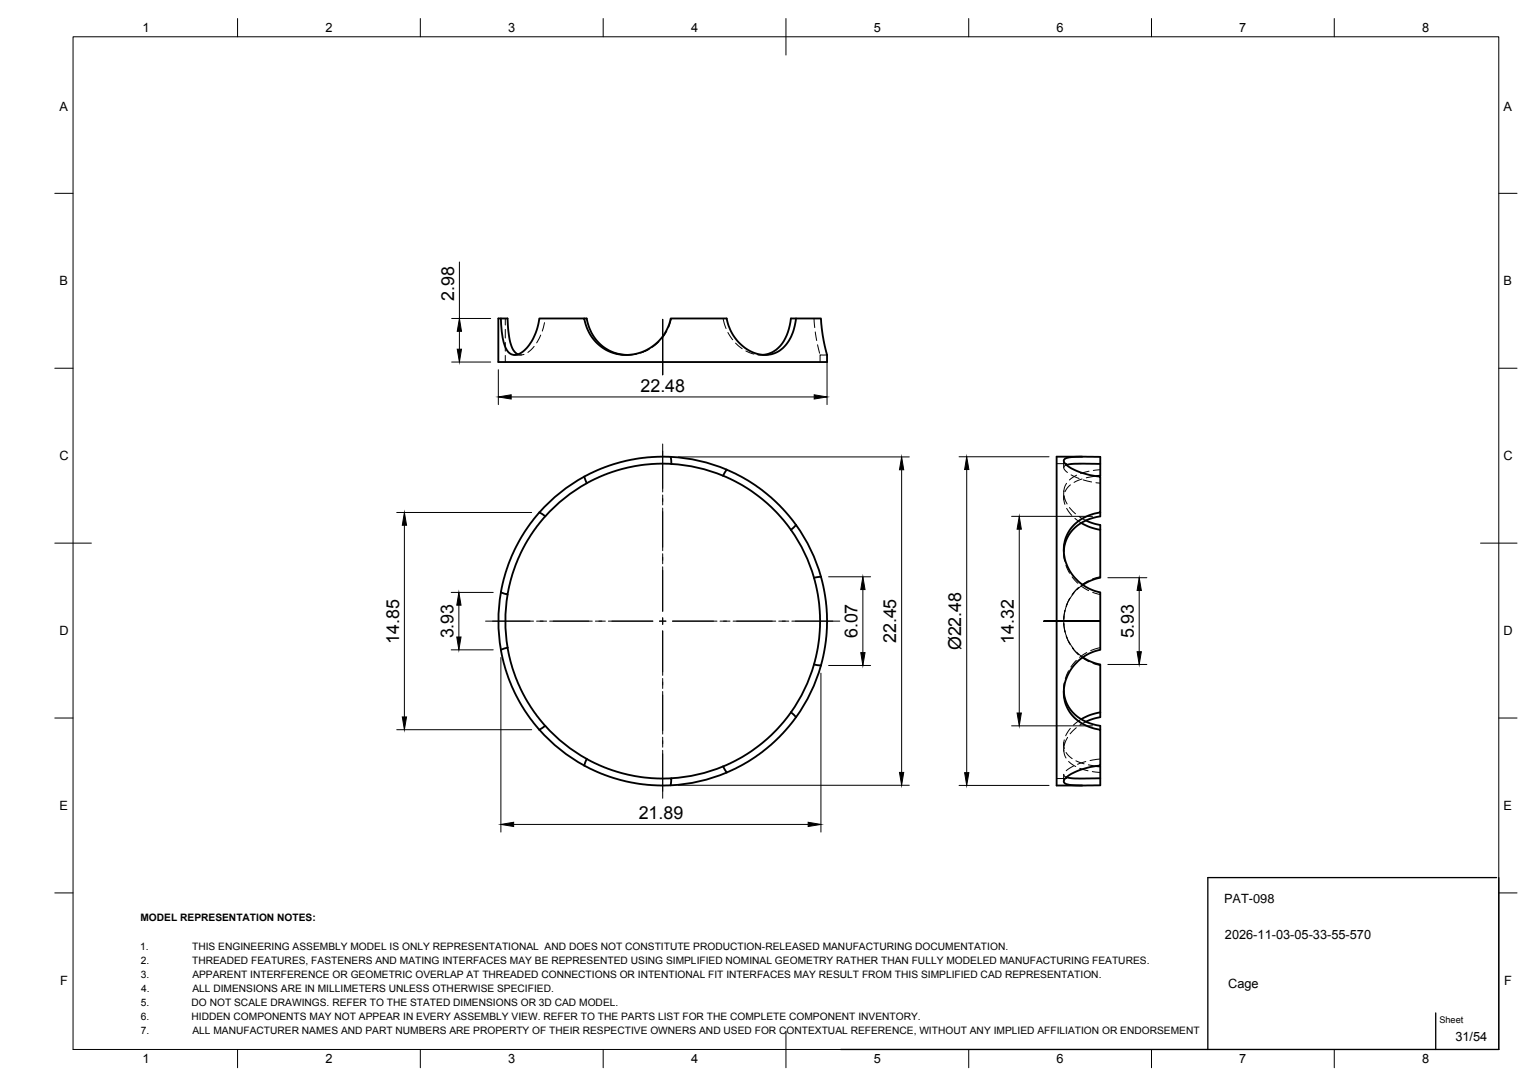
ISO-10303-21;
HEADER;
/* Generated by software containing ST-Developer
 * from STEP Tools, Inc. (www.steptools.com) 
 */

FILE_DESCRIPTION(
/* description */ ('Spring compression tester'),
/* implementation_level */ '2;1');

FILE_NAME(
/* name */ 'Cage.step',
/* time_stamp */ '2026-10-28T03:24:11-07:00',
/* author */ (''),
/* organization */ (''),
/* preprocessor_version */ 'ST-DEVELOPER v20.2',
/* originating_system */ 'Autodesk Translation Framework v15.17.0.0',
/* authorisation */ '');

FILE_SCHEMA (('AUTOMOTIVE_DESIGN { 1 0 10303 214 3 1 1 }'));
ENDSEC;

DATA;
#10=MECHANICAL_DESIGN_GEOMETRIC_PRESENTATION_REPRESENTATION('',(#1136),#43521);
#553=B_SPLINE_CURVE_WITH_KNOTS('',3,(#28592,#28593,#28594,#28595,#28596,
#28597,#28598,#28599,#28600,#28601,#28602,#28603,#28604,#28605,#28606,#28607,
#28608,#28609,#28610,#28611,#28612,#28613),.UNSPECIFIED.,.F.,.F.,(4,2,2,
2,2,2,2,2,2,2,4),(0.0591825211272536,0.157966726598481,0.236950089897721,
0.315933453196962,0.391576304923761,0.46721915665056,0.54286200837736,0.618504860104159,
0.697488223403399,0.77647158670264,0.875255792173867),.UNSPECIFIED.);
#554=B_SPLINE_CURVE_WITH_KNOTS('',3,(#28617,#28618,#28619,#28620,#28621,
#28622,#28623,#28624,#28625,#28626,#28627,#28628,#28629,#28630,#28631,#28632,
#28633,#28634,#28635,#28636,#28637,#28638),.UNSPECIFIED.,.F.,.F.,(4,2,2,
2,2,2,2,2,2,2,4),(0.0581119756758434,0.106553146291161,0.213106292582322,
0.30849933801665,0.386091982889075,0.4636846277615,0.541277272633925,0.61886991750635,
0.714262962940678,0.820816109231839,0.869257279847157),.UNSPECIFIED.);
#555=B_SPLINE_CURVE_WITH_KNOTS('',3,(#28644,#28645,#28646,#28647,#28648,
#28649,#28650,#28651,#28652,#28653,#28654,#28655,#28656,#28657,#28658,#28659,
#28660,#28661,#28662,#28663,#28664,#28665),.UNSPECIFIED.,.F.,.F.,(4,2,2,
2,2,2,2,2,2,2,4),(0.0581119756758434,0.106553146291161,0.213106292582322,
0.30849933801665,0.386091982889075,0.4636846277615,0.541277272633925,0.61886991750635,
0.714262962940679,0.820816109231839,0.869257279847157),.UNSPECIFIED.);
#556=B_SPLINE_CURVE_WITH_KNOTS('',3,(#28669,#28670,#28671,#28672,#28673,
#28674,#28675,#28676,#28677,#28678,#28679,#28680,#28681,#28682,#28683,#28684,
#28685,#28686,#28687,#28688,#28689,#28690),.UNSPECIFIED.,.F.,.F.,(4,2,2,
2,2,2,2,2,2,2,4),(0.0581119756758433,0.106553146291161,0.213106292582322,
0.308499338016649,0.386091982889075,0.4636846277615,0.541277272633925,0.61886991750635,
0.714262962940678,0.820816109231839,0.869257279847157),.UNSPECIFIED.);
#557=B_SPLINE_CURVE_WITH_KNOTS('',3,(#28699,#28700,#28701,#28702,#28703,
#28704,#28705,#28706,#28707,#28708,#28709,#28710,#28711,#28712,#28713,#28714,
#28715,#28716,#28717,#28718,#28719,#28720),.UNSPECIFIED.,.F.,.F.,(4,2,2,
2,2,2,2,2,2,2,4),(0.0581119756758433,0.106553146291161,0.213106292582322,
0.30849933801665,0.386091982889075,0.4636846277615,0.541277272633925,0.61886991750635,
0.714262962940678,0.820816109231839,0.869257279847157),.UNSPECIFIED.);
#558=B_SPLINE_CURVE_WITH_KNOTS('',3,(#28724,#28725,#28726,#28727,#28728,
#28729,#28730,#28731,#28732,#28733,#28734,#28735,#28736,#28737,#28738,#28739,
#28740,#28741,#28742,#28743,#28744,#28745),.UNSPECIFIED.,.F.,.F.,(4,2,2,
2,2,2,2,2,2,2,4),(0.0581119756758434,0.106553146291161,0.213106292582322,
0.30849933801665,0.386091982889075,0.4636846277615,0.541277272633925,0.61886991750635,
0.714262962940678,0.820816109231839,0.869257279847157),.UNSPECIFIED.);
#559=B_SPLINE_CURVE_WITH_KNOTS('',3,(#28749,#28750,#28751,#28752,#28753,
#28754,#28755,#28756,#28757,#28758,#28759,#28760,#28761,#28762,#28763,#28764,
#28765,#28766,#28767,#28768,#28769,#28770),.UNSPECIFIED.,.F.,.F.,(4,2,2,
2,2,2,2,2,2,2,4),(0.0581119756758434,0.106553146291161,0.213106292582322,
0.30849933801665,0.386091982889075,0.4636846277615,0.541277272633925,0.61886991750635,
0.714262962940678,0.820816109231839,0.869257279847157),.UNSPECIFIED.);
#560=B_SPLINE_CURVE_WITH_KNOTS('',3,(#28774,#28775,#28776,#28777,#28778,
#28779,#28780,#28781,#28782,#28783,#28784,#28785,#28786,#28787,#28788,#28789,
#28790,#28791,#28792,#28793,#28794,#28795),.UNSPECIFIED.,.F.,.F.,(4,2,2,
2,2,2,2,2,2,2,4),(0.0581119756758433,0.106553146291161,0.213106292582322,
0.30849933801665,0.386091982889075,0.4636846277615,0.541277272633925,0.61886991750635,
0.714262962940678,0.820816109231839,0.869257279847157),.UNSPECIFIED.);
#561=B_SPLINE_CURVE_WITH_KNOTS('',3,(#28803,#28804,#28805,#28806,#28807,
#28808,#28809,#28810,#28811,#28812,#28813,#28814,#28815,#28816,#28817,#28818,
#28819,#28820,#28821,#28822,#28823,#28824),.UNSPECIFIED.,.F.,.F.,(4,2,2,
2,2,2,2,2,2,2,4),(0.0591825211272536,0.157966726598481,0.236950089897721,
0.315933453196962,0.391576304923761,0.467219156650561,0.54286200837736,
0.618504860104159,0.697488223403399,0.77647158670264,0.875255792173867),
 .UNSPECIFIED.);
#562=B_SPLINE_CURVE_WITH_KNOTS('',3,(#28832,#28833,#28834,#28835,#28836,
#28837,#28838,#28839,#28840,#28841,#28842,#28843,#28844,#28845,#28846,#28847,
#28848,#28849,#28850,#28851,#28852,#28853),.UNSPECIFIED.,.F.,.F.,(4,2,2,
2,2,2,2,2,2,2,4),(0.0591825211272536,0.157966726598481,0.236950089897722,
0.315933453196962,0.391576304923761,0.467219156650561,0.54286200837736,
0.618504860104159,0.697488223403399,0.77647158670264,0.875255792173867),
 .UNSPECIFIED.);
#563=B_SPLINE_CURVE_WITH_KNOTS('',3,(#28863,#28864,#28865,#28866,#28867,
#28868,#28869,#28870,#28871,#28872,#28873,#28874,#28875,#28876,#28877,#28878,
#28879,#28880,#28881,#28882,#28883,#28884),.UNSPECIFIED.,.F.,.F.,(4,2,2,
2,2,2,2,2,2,2,4),(0.0591825211272536,0.157966726598481,0.236950089897721,
0.315933453196962,0.391576304923761,0.46721915665056,0.54286200837736,0.618504860104159,
0.697488223403399,0.77647158670264,0.875255792173867),.UNSPECIFIED.);
#564=B_SPLINE_CURVE_WITH_KNOTS('',3,(#28892,#28893,#28894,#28895,#28896,
#28897,#28898,#28899,#28900,#28901,#28902,#28903,#28904,#28905,#28906,#28907,
#28908,#28909,#28910,#28911,#28912,#28913),.UNSPECIFIED.,.F.,.F.,(4,2,2,
2,2,2,2,2,2,2,4),(0.0591825211272536,0.157966726598481,0.236950089897721,
0.315933453196962,0.391576304923761,0.46721915665056,0.542862008377359,
0.618504860104159,0.697488223403399,0.776471586702639,0.875255792173867),
 .UNSPECIFIED.);
#565=B_SPLINE_CURVE_WITH_KNOTS('',3,(#28921,#28922,#28923,#28924,#28925,
#28926,#28927,#28928,#28929,#28930,#28931,#28932,#28933,#28934,#28935,#28936,
#28937,#28938,#28939,#28940,#28941,#28942),.UNSPECIFIED.,.F.,.F.,(4,2,2,
2,2,2,2,2,2,2,4),(0.0591825211272536,0.157966726598481,0.236950089897721,
0.315933453196962,0.391576304923761,0.46721915665056,0.54286200837736,0.618504860104159,
0.697488223403399,0.77647158670264,0.875255792173867),.UNSPECIFIED.);
#566=B_SPLINE_CURVE_WITH_KNOTS('',3,(#28951,#28952,#28953,#28954,#28955,
#28956,#28957,#28958,#28959,#28960,#28961,#28962,#28963,#28964,#28965,#28966,
#28967,#28968,#28969,#28970,#28971,#28972),.UNSPECIFIED.,.F.,.F.,(4,2,2,
2,2,2,2,2,2,2,4),(0.0591825211272536,0.157966726598481,0.236950089897721,
0.315933453196962,0.391576304923761,0.46721915665056,0.542862008377359,
0.618504860104159,0.697488223403399,0.776471586702639,0.875255792173867),
 .UNSPECIFIED.);
#904=SPHERICAL_SURFACE('',#20049,0.309556);
#905=SPHERICAL_SURFACE('',#20065,0.309556);
#906=SPHERICAL_SURFACE('',#20070,0.309556);
#907=SPHERICAL_SURFACE('',#20076,0.309556);
#908=SPHERICAL_SURFACE('',#20081,0.309556);
#909=SPHERICAL_SURFACE('',#20086,0.309556);
#910=SPHERICAL_SURFACE('',#20094,0.309556);
#1010=SHAPE_REPRESENTATION_RELATIONSHIP('SRR','None',#43823,#1070);
#1070=ADVANCED_BREP_SHAPE_REPRESENTATION('',(#1210),#43483);
#1136=STYLED_ITEM('',(#44202),#1210);
#1210=MANIFOLD_SOLID_BREP('Continuous crown cage',#18574);
#1454=FACE_BOUND('',#3889,.T.);
#1892=PLANE('',#20062);
#1893=PLANE('',#20067);
#1894=PLANE('',#20072);
#1895=PLANE('',#20078);
#1896=PLANE('',#20083);
#1897=PLANE('',#20092);
#1898=PLANE('',#20096);
#1899=PLANE('',#20097);
#2619=FACE_OUTER_BOUND('',#3873,.T.);
#2620=FACE_OUTER_BOUND('',#3874,.T.);
#2621=FACE_OUTER_BOUND('',#3875,.T.);
#2622=FACE_OUTER_BOUND('',#3876,.T.);
#2623=FACE_OUTER_BOUND('',#3877,.T.);
#2624=FACE_OUTER_BOUND('',#3878,.T.);
#2625=FACE_OUTER_BOUND('',#3879,.T.);
#2626=FACE_OUTER_BOUND('',#3880,.T.);
#2627=FACE_OUTER_BOUND('',#3881,.T.);
#2628=FACE_OUTER_BOUND('',#3882,.T.);
#2629=FACE_OUTER_BOUND('',#3883,.T.);
#2630=FACE_OUTER_BOUND('',#3884,.T.);
#2631=FACE_OUTER_BOUND('',#3885,.T.);
#2632=FACE_OUTER_BOUND('',#3886,.T.);
#2633=FACE_OUTER_BOUND('',#3887,.T.);
#2634=FACE_OUTER_BOUND('',#3888,.T.);
#2635=FACE_OUTER_BOUND('',#3890,.T.);
#3873=EDGE_LOOP('',(#14199,#14200,#14201,#14202));
#3874=EDGE_LOOP('',(#14203,#14204,#14205,#14206,#14207,#14208,#14209,#14210,
#14211,#14212,#14213,#14214,#14215,#14216,#14217,#14218,#14219,#14220));
#3875=EDGE_LOOP('',(#14221,#14222,#14223,#14224));
#3876=EDGE_LOOP('',(#14225,#14226,#14227,#14228));
#3877=EDGE_LOOP('',(#14229,#14230,#14231,#14232));
#3878=EDGE_LOOP('',(#14233,#14234,#14235,#14236));
#3879=EDGE_LOOP('',(#14237,#14238,#14239,#14240,#14241,#14242));
#3880=EDGE_LOOP('',(#14243,#14244,#14245,#14246));
#3881=EDGE_LOOP('',(#14247,#14248,#14249,#14250));
#3882=EDGE_LOOP('',(#14251,#14252,#14253,#14254));
#3883=EDGE_LOOP('',(#14255,#14256,#14257,#14258));
#3884=EDGE_LOOP('',(#14259,#14260,#14261,#14262));
#3885=EDGE_LOOP('',(#14263,#14264,#14265,#14266,#14267,#14268,#14269,#14270,
#14271,#14272,#14273,#14274,#14275,#14276,#14277,#14278,#14279,#14280));
#3886=EDGE_LOOP('',(#14281,#14282,#14283,#14284));
#3887=EDGE_LOOP('',(#14285,#14286,#14287,#14288));
#3888=EDGE_LOOP('',(#14289));
#3889=EDGE_LOOP('',(#14290));
#3890=EDGE_LOOP('',(#14291,#14292,#14293,#14294));
#5311=LINE('',#28694,#6743);
#5312=LINE('',#28947,#6744);
#6743=VECTOR('',#23445,1.123812);
#6744=VECTOR('',#23514,1.076188);
#7756=CIRCLE('',#20050,0.303778037777585);
#7757=CIRCLE('',#20051,0.303778037777585);
#7758=CIRCLE('',#20053,1.123812);
#7759=CIRCLE('',#20054,1.123812);
#7760=CIRCLE('',#20055,1.123812);
#7761=CIRCLE('',#20056,1.123812);
#7762=CIRCLE('',#20057,1.123812);
#7763=CIRCLE('',#20058,1.123812);
#7764=CIRCLE('',#20059,1.123812);
#7765=CIRCLE('',#20060,1.123812);
#7766=CIRCLE('',#20061,1.123812);
#7767=CIRCLE('',#20063,1.076188);
#7768=CIRCLE('',#20064,0.303778037777585);
#7769=CIRCLE('',#20066,0.303778037777585);
#7770=CIRCLE('',#20068,1.076188);
#7771=CIRCLE('',#20069,0.303778037777585);
#7772=CIRCLE('',#20071,0.303778037777585);
#7773=CIRCLE('',#20073,1.076188);
#7774=CIRCLE('',#20074,1.076188);
#7775=CIRCLE('',#20075,0.303778037777585);
#7776=CIRCLE('',#20077,0.303778037777585);
#7777=CIRCLE('',#20079,1.076188);
#7778=CIRCLE('',#20080,0.303778037777585);
#7779=CIRCLE('',#20082,0.303778037777585);
#7780=CIRCLE('',#20084,1.076188);
#7781=CIRCLE('',#20085,0.303778037777585);
#7782=CIRCLE('',#20087,0.303778037777585);
#7783=CIRCLE('',#20089,1.076188);
#7784=CIRCLE('',#20090,1.076188);
#7785=CIRCLE('',#20091,1.076188);
#7786=CIRCLE('',#20093,0.303778037777585);
#7787=CIRCLE('',#20095,0.303778037777585);
#8803=VERTEX_POINT('',#28590);
#8804=VERTEX_POINT('',#28591);
#8805=VERTEX_POINT('',#28614);
#8806=VERTEX_POINT('',#28616);
#8807=VERTEX_POINT('',#28641);
#8808=VERTEX_POINT('',#28643);
#8809=VERTEX_POINT('',#28666);
#8810=VERTEX_POINT('',#28668);
#8811=VERTEX_POINT('',#28691);
#8812=VERTEX_POINT('',#28693);
#8813=VERTEX_POINT('',#28696);
#8814=VERTEX_POINT('',#28698);
#8815=VERTEX_POINT('',#28721);
#8816=VERTEX_POINT('',#28723);
#8817=VERTEX_POINT('',#28746);
#8818=VERTEX_POINT('',#28748);
#8819=VERTEX_POINT('',#28771);
#8820=VERTEX_POINT('',#28773);
#8821=VERTEX_POINT('',#28798);
#8822=VERTEX_POINT('',#28802);
#8823=VERTEX_POINT('',#28827);
#8824=VERTEX_POINT('',#28831);
#8825=VERTEX_POINT('',#28856);
#8826=VERTEX_POINT('',#28858);
#8827=VERTEX_POINT('',#28862);
#8828=VERTEX_POINT('',#28887);
#8829=VERTEX_POINT('',#28891);
#8830=VERTEX_POINT('',#28916);
#8831=VERTEX_POINT('',#28920);
#8832=VERTEX_POINT('',#28945);
#8833=VERTEX_POINT('',#28948);
#8834=VERTEX_POINT('',#28950);
#10764=EDGE_CURVE('',#8803,#8804,#553,.T.);
#10765=EDGE_CURVE('',#8805,#8803,#7756,.T.);
#10766=EDGE_CURVE('',#8806,#8805,#554,.T.);
#10767=EDGE_CURVE('',#8804,#8806,#7757,.T.);
#10768=EDGE_CURVE('',#8807,#8805,#7758,.T.);
#10769=EDGE_CURVE('',#8807,#8808,#555,.T.);
#10770=EDGE_CURVE('',#8809,#8808,#7759,.T.);
#10771=EDGE_CURVE('',#8809,#8810,#556,.T.);
#10772=EDGE_CURVE('',#8811,#8810,#7760,.T.);
#10773=EDGE_CURVE('',#8811,#8812,#5311,.T.);
#10774=EDGE_CURVE('',#8812,#8812,#7761,.T.);
#10775=EDGE_CURVE('',#8813,#8811,#7762,.T.);
#10776=EDGE_CURVE('',#8813,#8814,#557,.T.);
#10777=EDGE_CURVE('',#8815,#8814,#7763,.T.);
#10778=EDGE_CURVE('',#8815,#8816,#558,.T.);
#10779=EDGE_CURVE('',#8817,#8816,#7764,.T.);
#10780=EDGE_CURVE('',#8817,#8818,#559,.T.);
#10781=EDGE_CURVE('',#8819,#8818,#7765,.T.);
#10782=EDGE_CURVE('',#8819,#8820,#560,.T.);
#10783=EDGE_CURVE('',#8806,#8820,#7766,.T.);
#10784=EDGE_CURVE('',#8803,#8821,#7767,.T.);
#10785=EDGE_CURVE('',#8821,#8807,#7768,.T.);
#10786=EDGE_CURVE('',#8822,#8821,#561,.T.);
#10787=EDGE_CURVE('',#8808,#8822,#7769,.T.);
#10788=EDGE_CURVE('',#8822,#8823,#7770,.T.);
#10789=EDGE_CURVE('',#8823,#8809,#7771,.T.);
#10790=EDGE_CURVE('',#8824,#8823,#562,.T.);
#10791=EDGE_CURVE('',#8810,#8824,#7772,.T.);
#10792=EDGE_CURVE('',#8824,#8825,#7773,.T.);
#10793=EDGE_CURVE('',#8825,#8826,#7774,.T.);
#10794=EDGE_CURVE('',#8826,#8813,#7775,.T.);
#10795=EDGE_CURVE('',#8827,#8826,#563,.T.);
#10796=EDGE_CURVE('',#8814,#8827,#7776,.T.);
#10797=EDGE_CURVE('',#8827,#8828,#7777,.T.);
#10798=EDGE_CURVE('',#8828,#8815,#7778,.T.);
#10799=EDGE_CURVE('',#8829,#8828,#564,.T.);
#10800=EDGE_CURVE('',#8816,#8829,#7779,.T.);
#10801=EDGE_CURVE('',#8829,#8830,#7780,.T.);
#10802=EDGE_CURVE('',#8830,#8817,#7781,.T.);
#10803=EDGE_CURVE('',#8831,#8830,#565,.T.);
#10804=EDGE_CURVE('',#8818,#8831,#7782,.T.);
#10805=EDGE_CURVE('',#8832,#8832,#7783,.T.);
#10806=EDGE_CURVE('',#8832,#8825,#5312,.T.);
#10807=EDGE_CURVE('',#8833,#8804,#7784,.T.);
#10808=EDGE_CURVE('',#8833,#8834,#566,.T.);
#10809=EDGE_CURVE('',#8831,#8834,#7785,.T.);
#10810=EDGE_CURVE('',#8820,#8833,#7786,.T.);
#10811=EDGE_CURVE('',#8834,#8819,#7787,.T.);
#14199=ORIENTED_EDGE('',*,*,#10764,.F.);
#14200=ORIENTED_EDGE('',*,*,#10765,.F.);
#14201=ORIENTED_EDGE('',*,*,#10766,.F.);
#14202=ORIENTED_EDGE('',*,*,#10767,.F.);
#14203=ORIENTED_EDGE('',*,*,#10766,.T.);
#14204=ORIENTED_EDGE('',*,*,#10768,.F.);
#14205=ORIENTED_EDGE('',*,*,#10769,.T.);
#14206=ORIENTED_EDGE('',*,*,#10770,.F.);
#14207=ORIENTED_EDGE('',*,*,#10771,.T.);
#14208=ORIENTED_EDGE('',*,*,#10772,.F.);
#14209=ORIENTED_EDGE('',*,*,#10773,.T.);
#14210=ORIENTED_EDGE('',*,*,#10774,.F.);
#14211=ORIENTED_EDGE('',*,*,#10773,.F.);
#14212=ORIENTED_EDGE('',*,*,#10775,.F.);
#14213=ORIENTED_EDGE('',*,*,#10776,.T.);
#14214=ORIENTED_EDGE('',*,*,#10777,.F.);
#14215=ORIENTED_EDGE('',*,*,#10778,.T.);
#14216=ORIENTED_EDGE('',*,*,#10779,.F.);
#14217=ORIENTED_EDGE('',*,*,#10780,.T.);
#14218=ORIENTED_EDGE('',*,*,#10781,.F.);
#14219=ORIENTED_EDGE('',*,*,#10782,.T.);
#14220=ORIENTED_EDGE('',*,*,#10783,.F.);
#14221=ORIENTED_EDGE('',*,*,#10765,.T.);
#14222=ORIENTED_EDGE('',*,*,#10784,.T.);
#14223=ORIENTED_EDGE('',*,*,#10785,.T.);
#14224=ORIENTED_EDGE('',*,*,#10768,.T.);
#14225=ORIENTED_EDGE('',*,*,#10786,.F.);
#14226=ORIENTED_EDGE('',*,*,#10787,.F.);
#14227=ORIENTED_EDGE('',*,*,#10769,.F.);
#14228=ORIENTED_EDGE('',*,*,#10785,.F.);
#14229=ORIENTED_EDGE('',*,*,#10787,.T.);
#14230=ORIENTED_EDGE('',*,*,#10788,.T.);
#14231=ORIENTED_EDGE('',*,*,#10789,.T.);
#14232=ORIENTED_EDGE('',*,*,#10770,.T.);
#14233=ORIENTED_EDGE('',*,*,#10790,.F.);
#14234=ORIENTED_EDGE('',*,*,#10791,.F.);
#14235=ORIENTED_EDGE('',*,*,#10771,.F.);
#14236=ORIENTED_EDGE('',*,*,#10789,.F.);
#14237=ORIENTED_EDGE('',*,*,#10791,.T.);
#14238=ORIENTED_EDGE('',*,*,#10792,.T.);
#14239=ORIENTED_EDGE('',*,*,#10793,.T.);
#14240=ORIENTED_EDGE('',*,*,#10794,.T.);
#14241=ORIENTED_EDGE('',*,*,#10775,.T.);
#14242=ORIENTED_EDGE('',*,*,#10772,.T.);
#14243=ORIENTED_EDGE('',*,*,#10795,.F.);
#14244=ORIENTED_EDGE('',*,*,#10796,.F.);
#14245=ORIENTED_EDGE('',*,*,#10776,.F.);
#14246=ORIENTED_EDGE('',*,*,#10794,.F.);
#14247=ORIENTED_EDGE('',*,*,#10796,.T.);
#14248=ORIENTED_EDGE('',*,*,#10797,.T.);
#14249=ORIENTED_EDGE('',*,*,#10798,.T.);
#14250=ORIENTED_EDGE('',*,*,#10777,.T.);
#14251=ORIENTED_EDGE('',*,*,#10799,.F.);
#14252=ORIENTED_EDGE('',*,*,#10800,.F.);
#14253=ORIENTED_EDGE('',*,*,#10778,.F.);
#14254=ORIENTED_EDGE('',*,*,#10798,.F.);
#14255=ORIENTED_EDGE('',*,*,#10800,.T.);
#14256=ORIENTED_EDGE('',*,*,#10801,.T.);
#14257=ORIENTED_EDGE('',*,*,#10802,.T.);
#14258=ORIENTED_EDGE('',*,*,#10779,.T.);
#14259=ORIENTED_EDGE('',*,*,#10780,.F.);
#14260=ORIENTED_EDGE('',*,*,#10802,.F.);
#14261=ORIENTED_EDGE('',*,*,#10803,.F.);
#14262=ORIENTED_EDGE('',*,*,#10804,.F.);
#14263=ORIENTED_EDGE('',*,*,#10805,.F.);
#14264=ORIENTED_EDGE('',*,*,#10806,.T.);
#14265=ORIENTED_EDGE('',*,*,#10792,.F.);
#14266=ORIENTED_EDGE('',*,*,#10790,.T.);
#14267=ORIENTED_EDGE('',*,*,#10788,.F.);
#14268=ORIENTED_EDGE('',*,*,#10786,.T.);
#14269=ORIENTED_EDGE('',*,*,#10784,.F.);
#14270=ORIENTED_EDGE('',*,*,#10764,.T.);
#14271=ORIENTED_EDGE('',*,*,#10807,.F.);
#14272=ORIENTED_EDGE('',*,*,#10808,.T.);
#14273=ORIENTED_EDGE('',*,*,#10809,.F.);
#14274=ORIENTED_EDGE('',*,*,#10803,.T.);
#14275=ORIENTED_EDGE('',*,*,#10801,.F.);
#14276=ORIENTED_EDGE('',*,*,#10799,.T.);
#14277=ORIENTED_EDGE('',*,*,#10797,.F.);
#14278=ORIENTED_EDGE('',*,*,#10795,.T.);
#14279=ORIENTED_EDGE('',*,*,#10793,.F.);
#14280=ORIENTED_EDGE('',*,*,#10806,.F.);
#14281=ORIENTED_EDGE('',*,*,#10767,.T.);
#14282=ORIENTED_EDGE('',*,*,#10783,.T.);
#14283=ORIENTED_EDGE('',*,*,#10810,.T.);
#14284=ORIENTED_EDGE('',*,*,#10807,.T.);
#14285=ORIENTED_EDGE('',*,*,#10782,.F.);
#14286=ORIENTED_EDGE('',*,*,#10811,.F.);
#14287=ORIENTED_EDGE('',*,*,#10808,.F.);
#14288=ORIENTED_EDGE('',*,*,#10810,.F.);
#14289=ORIENTED_EDGE('',*,*,#10774,.T.);
#14290=ORIENTED_EDGE('',*,*,#10805,.T.);
#14291=ORIENTED_EDGE('',*,*,#10804,.T.);
#14292=ORIENTED_EDGE('',*,*,#10809,.T.);
#14293=ORIENTED_EDGE('',*,*,#10811,.T.);
#14294=ORIENTED_EDGE('',*,*,#10781,.T.);
#17233=CYLINDRICAL_SURFACE('',#20052,1.123812);
#17234=CYLINDRICAL_SURFACE('',#20088,1.076188);
#17943=ADVANCED_FACE('',(#2619),#904,.F.);
#17944=ADVANCED_FACE('',(#2620),#17233,.T.);
#17945=ADVANCED_FACE('',(#2621),#1892,.T.);
#17946=ADVANCED_FACE('',(#2622),#905,.F.);
#17947=ADVANCED_FACE('',(#2623),#1893,.T.);
#17948=ADVANCED_FACE('',(#2624),#906,.F.);
#17949=ADVANCED_FACE('',(#2625),#1894,.T.);
#17950=ADVANCED_FACE('',(#2626),#907,.F.);
#17951=ADVANCED_FACE('',(#2627),#1895,.T.);
#17952=ADVANCED_FACE('',(#2628),#908,.F.);
#17953=ADVANCED_FACE('',(#2629),#1896,.T.);
#17954=ADVANCED_FACE('',(#2630),#909,.F.);
#17955=ADVANCED_FACE('',(#2631),#17234,.F.);
#17956=ADVANCED_FACE('',(#2632),#1897,.T.);
#17957=ADVANCED_FACE('',(#2633),#910,.F.);
#17958=ADVANCED_FACE('',(#2634,#1454),#1898,.T.);
#17959=ADVANCED_FACE('',(#2635),#1899,.T.);
#18574=CLOSED_SHELL('',(#17943,#17944,#17945,#17946,#17947,#17948,#17949,
#17950,#17951,#17952,#17953,#17954,#17955,#17956,#17957,#17958,#17959));
#20048=AXIS2_PLACEMENT_3D('',#28588,#23429,#23430);
#20049=AXIS2_PLACEMENT_3D('',#28589,#23431,#23432);
#20050=AXIS2_PLACEMENT_3D('',#28615,#23433,#23434);
#20051=AXIS2_PLACEMENT_3D('',#28639,#23435,#23436);
#20052=AXIS2_PLACEMENT_3D('',#28640,#23437,#23438);
#20053=AXIS2_PLACEMENT_3D('',#28642,#23439,#23440);
#20054=AXIS2_PLACEMENT_3D('',#28667,#23441,#23442);
#20055=AXIS2_PLACEMENT_3D('',#28692,#23443,#23444);
#20056=AXIS2_PLACEMENT_3D('',#28695,#23446,#23447);
#20057=AXIS2_PLACEMENT_3D('',#28697,#23448,#23449);
#20058=AXIS2_PLACEMENT_3D('',#28722,#23450,#23451);
#20059=AXIS2_PLACEMENT_3D('',#28747,#23452,#23453);
#20060=AXIS2_PLACEMENT_3D('',#28772,#23454,#23455);
#20061=AXIS2_PLACEMENT_3D('',#28796,#23456,#23457);
#20062=AXIS2_PLACEMENT_3D('',#28797,#23458,#23459);
#20063=AXIS2_PLACEMENT_3D('',#28799,#23460,#23461);
#20064=AXIS2_PLACEMENT_3D('',#28800,#23462,#23463);
#20065=AXIS2_PLACEMENT_3D('',#28801,#23464,#23465);
#20066=AXIS2_PLACEMENT_3D('',#28825,#23466,#23467);
#20067=AXIS2_PLACEMENT_3D('',#28826,#23468,#23469);
#20068=AXIS2_PLACEMENT_3D('',#28828,#23470,#23471);
#20069=AXIS2_PLACEMENT_3D('',#28829,#23472,#23473);
#20070=AXIS2_PLACEMENT_3D('',#28830,#23474,#23475);
#20071=AXIS2_PLACEMENT_3D('',#28854,#23476,#23477);
#20072=AXIS2_PLACEMENT_3D('',#28855,#23478,#23479);
#20073=AXIS2_PLACEMENT_3D('',#28857,#23480,#23481);
#20074=AXIS2_PLACEMENT_3D('',#28859,#23482,#23483);
#20075=AXIS2_PLACEMENT_3D('',#28860,#23484,#23485);
#20076=AXIS2_PLACEMENT_3D('',#28861,#23486,#23487);
#20077=AXIS2_PLACEMENT_3D('',#28885,#23488,#23489);
#20078=AXIS2_PLACEMENT_3D('',#28886,#23490,#23491);
#20079=AXIS2_PLACEMENT_3D('',#28888,#23492,#23493);
#20080=AXIS2_PLACEMENT_3D('',#28889,#23494,#23495);
#20081=AXIS2_PLACEMENT_3D('',#28890,#23496,#23497);
#20082=AXIS2_PLACEMENT_3D('',#28914,#23498,#23499);
#20083=AXIS2_PLACEMENT_3D('',#28915,#23500,#23501);
#20084=AXIS2_PLACEMENT_3D('',#28917,#23502,#23503);
#20085=AXIS2_PLACEMENT_3D('',#28918,#23504,#23505);
#20086=AXIS2_PLACEMENT_3D('',#28919,#23506,#23507);
#20087=AXIS2_PLACEMENT_3D('',#28943,#23508,#23509);
#20088=AXIS2_PLACEMENT_3D('',#28944,#23510,#23511);
#20089=AXIS2_PLACEMENT_3D('',#28946,#23512,#23513);
#20090=AXIS2_PLACEMENT_3D('',#28949,#23515,#23516);
#20091=AXIS2_PLACEMENT_3D('',#28973,#23517,#23518);
#20092=AXIS2_PLACEMENT_3D('',#28974,#23519,#23520);
#20093=AXIS2_PLACEMENT_3D('',#28975,#23521,#23522);
#20094=AXIS2_PLACEMENT_3D('',#28976,#23523,#23524);
#20095=AXIS2_PLACEMENT_3D('',#28977,#23525,#23526);
#20096=AXIS2_PLACEMENT_3D('',#28978,#23527,#23528);
#20097=AXIS2_PLACEMENT_3D('',#28979,#23529,#23530);
#23429=DIRECTION('axis',(0.,0.,1.));
#23430=DIRECTION('refdir',(1.,0.,0.));
#23431=DIRECTION('center_axis',(0.,0.,1.));
#23432=DIRECTION('ref_axis',(1.,0.,0.));
#23433=DIRECTION('center_axis',(0.,-1.,0.));
#23434=DIRECTION('ref_axis',(0.,0.,-1.));
#23435=DIRECTION('center_axis',(0.,-1.,0.));
#23436=DIRECTION('ref_axis',(0.,0.,-1.));
#23437=DIRECTION('center_axis',(0.,1.,0.));
#23438=DIRECTION('ref_axis',(1.,0.,0.));
#23439=DIRECTION('center_axis',(0.,1.,0.));
#23440=DIRECTION('ref_axis',(1.,0.,0.));
#23441=DIRECTION('center_axis',(0.,1.,0.));
#23442=DIRECTION('ref_axis',(1.,0.,0.));
#23443=DIRECTION('center_axis',(0.,1.,0.));
#23444=DIRECTION('ref_axis',(1.,0.,0.));
#23445=DIRECTION('',(0.,-1.,0.));
#23446=DIRECTION('center_axis',(0.,-1.,0.));
#23447=DIRECTION('ref_axis',(1.,0.,0.));
#23448=DIRECTION('center_axis',(0.,1.,0.));
#23449=DIRECTION('ref_axis',(1.,0.,0.));
#23450=DIRECTION('center_axis',(0.,1.,0.));
#23451=DIRECTION('ref_axis',(1.,0.,0.));
#23452=DIRECTION('center_axis',(0.,1.,0.));
#23453=DIRECTION('ref_axis',(1.,0.,0.));
#23454=DIRECTION('center_axis',(0.,1.,0.));
#23455=DIRECTION('ref_axis',(1.,0.,0.));
#23456=DIRECTION('center_axis',(0.,1.,0.));
#23457=DIRECTION('ref_axis',(1.,0.,0.));
#23458=DIRECTION('center_axis',(0.,1.,0.));
#23459=DIRECTION('ref_axis',(1.,0.,0.));
#23460=DIRECTION('center_axis',(0.,-1.,0.));
#23461=DIRECTION('ref_axis',(1.,0.,0.));
#23462=DIRECTION('center_axis',(0.,-1.,0.));
#23463=DIRECTION('ref_axis',(0.,0.,-1.));
#23464=DIRECTION('center_axis',(8.96625347776458E-17,0.,1.));
#23465=DIRECTION('ref_axis',(1.,0.,0.));
#23466=DIRECTION('center_axis',(0.,-1.,0.));
#23467=DIRECTION('ref_axis',(0.,0.,-1.));
#23468=DIRECTION('center_axis',(0.,1.,0.));
#23469=DIRECTION('ref_axis',(1.,0.,0.));
#23470=DIRECTION('center_axis',(0.,-1.,0.));
#23471=DIRECTION('ref_axis',(1.,0.,0.));
#23472=DIRECTION('center_axis',(0.,-1.,0.));
#23473=DIRECTION('ref_axis',(0.,0.,-1.));
#23474=DIRECTION('center_axis',(0.,0.,1.));
#23475=DIRECTION('ref_axis',(1.,0.,0.));
#23476=DIRECTION('center_axis',(0.,-1.,0.));
#23477=DIRECTION('ref_axis',(0.,0.,-1.));
#23478=DIRECTION('center_axis',(0.,1.,0.));
#23479=DIRECTION('ref_axis',(1.,0.,0.));
#23480=DIRECTION('center_axis',(0.,-1.,0.));
#23481=DIRECTION('ref_axis',(1.,0.,0.));
#23482=DIRECTION('center_axis',(0.,-1.,0.));
#23483=DIRECTION('ref_axis',(1.,0.,0.));
#23484=DIRECTION('center_axis',(0.,-1.,0.));
#23485=DIRECTION('ref_axis',(0.,0.,-1.));
#23486=DIRECTION('center_axis',(0.,0.,1.));
#23487=DIRECTION('ref_axis',(1.,0.,0.));
#23488=DIRECTION('center_axis',(0.,-1.,0.));
#23489=DIRECTION('ref_axis',(0.,0.,-1.));
#23490=DIRECTION('center_axis',(0.,1.,0.));
#23491=DIRECTION('ref_axis',(1.,0.,0.));
#23492=DIRECTION('center_axis',(0.,-1.,0.));
#23493=DIRECTION('ref_axis',(1.,0.,0.));
#23494=DIRECTION('center_axis',(0.,-1.,0.));
#23495=DIRECTION('ref_axis',(0.,0.,-1.));
#23496=DIRECTION('center_axis',(8.96625347776458E-17,0.,1.));
#23497=DIRECTION('ref_axis',(1.,0.,0.));
#23498=DIRECTION('center_axis',(0.,-1.,0.));
#23499=DIRECTION('ref_axis',(0.,0.,-1.));
#23500=DIRECTION('center_axis',(0.,1.,0.));
#23501=DIRECTION('ref_axis',(1.,0.,0.));
#23502=DIRECTION('center_axis',(0.,-1.,0.));
#23503=DIRECTION('ref_axis',(1.,0.,0.));
#23504=DIRECTION('center_axis',(0.,-1.,0.));
#23505=DIRECTION('ref_axis',(0.,0.,-1.));
#23506=DIRECTION('center_axis',(0.,0.,1.));
#23507=DIRECTION('ref_axis',(1.,0.,0.));
#23508=DIRECTION('center_axis',(0.,-1.,0.));
#23509=DIRECTION('ref_axis',(0.,0.,-1.));
#23510=DIRECTION('center_axis',(0.,1.,0.));
#23511=DIRECTION('ref_axis',(1.,0.,0.));
#23512=DIRECTION('center_axis',(0.,1.,0.));
#23513=DIRECTION('ref_axis',(1.,0.,0.));
#23514=DIRECTION('',(0.,1.,0.));
#23515=DIRECTION('center_axis',(0.,-1.,0.));
#23516=DIRECTION('ref_axis',(1.,0.,0.));
#23517=DIRECTION('center_axis',(0.,-1.,0.));
#23518=DIRECTION('ref_axis',(1.,0.,0.));
#23519=DIRECTION('center_axis',(0.,1.,0.));
#23520=DIRECTION('ref_axis',(1.,0.,0.));
#23521=DIRECTION('center_axis',(0.,-1.,0.));
#23522=DIRECTION('ref_axis',(0.,0.,-1.));
#23523=DIRECTION('center_axis',(0.,0.,1.));
#23524=DIRECTION('ref_axis',(1.,0.,0.));
#23525=DIRECTION('center_axis',(0.,-1.,0.));
#23526=DIRECTION('ref_axis',(0.,0.,-1.));
#23527=DIRECTION('center_axis',(0.,-1.,0.));
#23528=DIRECTION('ref_axis',(-1.,0.,0.));
#23529=DIRECTION('center_axis',(0.,1.,0.));
#23530=DIRECTION('ref_axis',(1.,0.,0.));
#28588=CARTESIAN_POINT('',(0.,0.,0.));
#28589=CARTESIAN_POINT('Origin',(0.685838782044607,0.,0.860014630714833));
#28590=CARTESIAN_POINT('',(0.413083465285518,-0.05953,0.993751811093549));
#28591=CARTESIAN_POINT('',(0.876916659919095,-0.05953,0.623857181492959));
#28592=CARTESIAN_POINT('Ctrl Pts',(0.413083465285518,-0.05953,0.993751811093549));
#28593=CARTESIAN_POINT('Ctrl Pts',(0.419070565453383,-0.0925528133349865,
0.991263089003441));
#28594=CARTESIAN_POINT('Ctrl Pts',(0.430199341854858,-0.124911173756694,
0.986608710139579));
#28595=CARTESIAN_POINT('Ctrl Pts',(0.457978755888596,-0.177924977804098,
0.973971221090534));
#28596=CARTESIAN_POINT('Ctrl Pts',(0.473077587363685,-0.199697230012983,
0.966820759530997));
#28597=CARTESIAN_POINT('Ctrl Pts',(0.507057380724533,-0.237895043532788,
0.949440676105255));
#28598=CARTESIAN_POINT('Ctrl Pts',(0.525933334162555,-0.254319232363049,
0.939198248544428));
#28599=CARTESIAN_POINT('Ctrl Pts',(0.564362943424238,-0.28018331644634,
0.916597376014514));
#28600=CARTESIAN_POINT('Ctrl Pts',(0.585840553788742,-0.29104845371857,
0.903141581680914));
#28601=CARTESIAN_POINT('Ctrl Pts',(0.629305439856167,-0.30527573347708,
0.873412008702649));
#28602=CARTESIAN_POINT('Ctrl Pts',(0.651278921914856,-0.308638795020976,
0.857118508332695));
#28603=CARTESIAN_POINT('Ctrl Pts',(0.690705563850638,-0.308638795020976,
0.825676810575914));
#28604=CARTESIAN_POINT('Ctrl Pts',(0.711480111898423,-0.30527573347708,
0.807879894508811));
#28605=CARTESIAN_POINT('Ctrl Pts',(0.750136149454208,-0.29104845371857,
0.772120216227122));
#28606=CARTESIAN_POINT('Ctrl Pts',(0.768033796848072,-0.28018331644634,
0.754175290318038));
#28607=CARTESIAN_POINT('Ctrl Pts',(0.798619410861634,-0.254319232363049,
0.721738358858166));
#28608=CARTESIAN_POINT('Ctrl Pts',(0.812805334167529,-0.237895043532788,
0.705614819529209));
#28609=CARTESIAN_POINT('Ctrl Pts',(0.837310877969633,-0.199697230012983,
0.676354402927683));
#28610=CARTESIAN_POINT('Ctrl Pts',(0.847641868610495,-0.177924977804098,
0.663225258065736));
#28611=CARTESIAN_POINT('Ctrl Pts',(0.866144010579847,-0.124911173756694,
0.638954437806245));
#28612=CARTESIAN_POINT('Ctrl Pts',(0.873158080166742,-0.0925528133349865,
0.62914037979579));
#28613=CARTESIAN_POINT('Ctrl Pts',(0.876916659919095,-0.05953,0.623857181492959));
#28614=CARTESIAN_POINT('',(0.437601487681057,-0.05953,1.03511272300331));
#28615=CARTESIAN_POINT('Origin',(0.685838782044607,-0.05953,0.860014630714833));
#28616=CARTESIAN_POINT('',(0.911784794170997,-0.05953,0.656964154625313));
#28617=CARTESIAN_POINT('Ctrl Pts',(0.911784794170998,-0.0595300000000001,
0.656964154625312));
#28618=CARTESIAN_POINT('Ctrl Pts',(0.909827729890942,-0.0762225747374255,
0.659680317203144));
#28619=CARTESIAN_POINT('Ctrl Pts',(0.907004864562642,-0.0928409665394228,
0.663576540841106));
#28620=CARTESIAN_POINT('Ctrl Pts',(0.895234408667242,-0.144299303100741,
0.679480524217551));
#28621=CARTESIAN_POINT('Ctrl Pts',(0.882797231409153,-0.177024326825049,
0.695831250979106));
#28622=CARTESIAN_POINT('Ctrl Pts',(0.854332839576145,-0.227269801620064,
0.73042219438957));
#28623=CARTESIAN_POINT('Ctrl Pts',(0.834863020612702,-0.251265615809407,
0.752807465209441));
#28624=CARTESIAN_POINT('Ctrl Pts',(0.800439809856111,-0.279889827963178,
0.789147407129766));
#28625=CARTESIAN_POINT('Ctrl Pts',(0.781998747691871,-0.290879136862659,
0.80756613568454));
#28626=CARTESIAN_POINT('Ctrl Pts',(0.742239891936898,-0.305251990234487,
0.844254137480382));
#28627=CARTESIAN_POINT('Ctrl Pts',(0.720906778729541,-0.308638795020976,
0.862505527716294));
#28628=CARTESIAN_POINT('Ctrl Pts',(0.680463863683392,-0.308638795020976,
0.894757676234429));
#28629=CARTESIAN_POINT('Ctrl Pts',(0.657923009631182,-0.305251990234488,
0.91149460735272));
#28630=CARTESIAN_POINT('Ctrl Pts',(0.613307674922609,-0.290879136862659,
0.942092777160053));
#28631=CARTESIAN_POINT('Ctrl Pts',(0.591247219971725,-0.279889827963178,
0.955972930713954));
#28632=CARTESIAN_POINT('Ctrl Pts',(0.548158511259202,-0.251265615809407,
0.981446681891443));
#28633=CARTESIAN_POINT('Ctrl Pts',(0.522002043615455,-0.227269801620063,
0.995447160474328));
#28634=CARTESIAN_POINT('Ctrl Pts',(0.481944444320713,-0.177024326825049,
1.01550068154148));
#28635=CARTESIAN_POINT('Ctrl Pts',(0.463236132117164,-0.14429930310074,
1.0239876538093));
#28636=CARTESIAN_POINT('Ctrl Pts',(0.445111721969657,-0.0928409665394226,
1.03192403056628));
#28637=CARTESIAN_POINT('Ctrl Pts',(0.440685038163619,-0.0762225747374254,
1.03380912944435));
#28638=CARTESIAN_POINT('Ctrl Pts',(0.437601487681056,-0.05953,1.03511272300331));
#28639=CARTESIAN_POINT('Origin',(0.685838782044607,-0.05953,0.860014630714833));
#28640=CARTESIAN_POINT('Origin',(0.,-0.208355,0.));
#28641=CARTESIAN_POINT('',(0.0548532617164168,-0.05953,1.12247250791415));
#28642=CARTESIAN_POINT('Origin',(0.,-0.05953,0.));
#28643=CARTESIAN_POINT('',(-0.536443649899848,-0.05953,0.987512846410683));
#28644=CARTESIAN_POINT('Ctrl Pts',(0.0548532617164173,-0.0595300000000001,
1.12247250791414));
#28645=CARTESIAN_POINT('Ctrl Pts',(0.05150947068137,-0.0762225747374254,
1.12263591311425));
#28646=CARTESIAN_POINT('Ctrl Pts',(0.0467032526342597,-0.0928409665394227,
1.12285816383385));
#28647=CARTESIAN_POINT('Ctrl Pts',(0.0269302585198975,-0.144299303100741,
1.12357162229597));
#28648=CARTESIAN_POINT('Ctrl Pts',(0.006392292392153,-0.177024326825049,
1.12404235695137));
#28649=CARTESIAN_POINT('Ctrl Pts',(-0.0383992541984087,-0.227269801620063,
1.12335509974011));
#28650=CARTESIAN_POINT('Ctrl Pts',(-0.0680399972366993,-0.251265615809407,
1.12208997038458));
#28651=CARTESIAN_POINT('Ctrl Pts',(-0.117914228755037,-0.279889827963178,
1.1178344036749));
#28652=CARTESIAN_POINT('Ctrl Pts',(-0.14381238480104,-0.290879136862659,
1.11490049012186));
#28653=CARTESIAN_POINT('Ctrl Pts',(-0.19728546073067,-0.305251990234488,
1.10669035995599));
#28654=CARTESIAN_POINT('Ctrl Pts',(-0.224855950742601,-0.308638795020976,
1.10139101611326));
#28655=CARTESIAN_POINT('Ctrl Pts',(-0.275287440920027,-0.308638795020976,
1.0898803575765));
#28656=CARTESIAN_POINT('Ctrl Pts',(-0.302426893214945,-0.305251990234488,
1.08269251410343));
#28657=CARTESIAN_POINT('Ctrl Pts',(-0.35416671187353,-0.290879136862659,
1.06688848765783));
#28658=CARTESIAN_POINT('Ctrl Pts',(-0.3787731215897,-0.279889827963178,
1.05829506364875));
#28659=CARTESIAN_POINT('Ctrl Pts',(-0.425554672694338,-0.251265615809407,
1.04048957871266));
#28660=CARTESIAN_POINT('Ctrl Pts',(-0.452808978448581,-0.227269801620063,
1.02876878445619));
#28661=CARTESIAN_POINT('Ctrl Pts',(-0.493462957200432,-0.177024326825049,
1.0099536580922));
#28662=CARTESIAN_POINT('Ctrl Pts',(-0.511762781179148,-0.14429930310074,
1.00061845128527));
#28663=CARTESIAN_POINT('Ctrl Pts',(-0.529268075276157,-0.0928409665394226,
0.991396466802468));
#28664=CARTESIAN_POINT('Ctrl Pts',(-0.533501897135713,-0.0762225747374254,
0.989110885965947));
#28665=CARTESIAN_POINT('Ctrl Pts',(-0.536443649899848,-0.0595300000000001,
0.987512846410683));
#28666=CARTESIAN_POINT('',(-0.843383895613249,-0.05953,0.742736168477219));
#28667=CARTESIAN_POINT('Origin',(0.,-0.05953,0.));
#28668=CARTESIAN_POINT('',(-1.10653577764992,-0.05953,0.196295654879792));
#28669=CARTESIAN_POINT('Ctrl Pts',(-0.843383895613249,-0.0595300000000001,
0.742736168477219));
#28670=CARTESIAN_POINT('Ctrl Pts',(-0.84559647055299,-0.0762225747374255,
0.740223768851062));
#28671=CARTESIAN_POINT('Ctrl Pts',(-0.848766861100456,-0.0928409665394227,
0.736604687327351));
#28672=CARTESIAN_POINT('Ctrl Pts',(-0.861652925570091,-0.144299303100741,
0.721590372101268));
#28673=CARTESIAN_POINT('Ctrl Pts',(-0.87482617317514,-0.177024326825049,
0.705826641853758));
#28674=CARTESIAN_POINT('Ctrl Pts',(-0.902215926359523,-0.227269801620063,
0.670378702718353));
#28675=CARTESIAN_POINT('Ctrl Pts',(-0.919707509403859,-0.251265615809407,
0.646415841396062));
#28676=CARTESIAN_POINT('Ctrl Pts',(-0.947476448101718,-0.279889827963178,
0.604769294586516));
#28677=CARTESIAN_POINT('Ctrl Pts',(-0.961329858300736,-0.290879136862659,
0.582692035672022));
#28678=CARTESIAN_POINT('Ctrl Pts',(-0.988250837578047,-0.305251990234488,
0.535766169015486));
#28679=CARTESIAN_POINT('Ctrl Pts',(-1.00129756308006,-0.308638795020976,
0.510906605094603));
#28680=CARTESIAN_POINT('Ctrl Pts',(-1.02374168767024,-0.308638795020976,
0.46430090015576));
#28681=CARTESIAN_POINT('Ctrl Pts',(-1.03504317708586,-0.305251990234488,
0.438600874831839));
#28682=CARTESIAN_POINT('Ctrl Pts',(-1.05494634094458,-0.290879136862659,
0.388295406390235));
#28683=CARTESIAN_POINT('Ctrl Pts',(-1.06356957703048,-0.279889827963178,
0.363699428370917));
#28684=CARTESIAN_POINT('Ctrl Pts',(-1.0788165083757,-0.251265615809407,
0.316022600643821));
#28685=CARTESIAN_POINT('Ctrl Pts',(-1.08664560412098,-0.227269801620063,
0.287406530683752));
#28686=CARTESIAN_POINT('Ctrl Pts',(-1.09728268713976,-0.177024326825049,
0.243890930799337));
#28687=CARTESIAN_POINT('Ctrl Pts',(-1.10139388218929,-0.144299303100741,
0.22376314604679));
#28688=CARTESIAN_POINT('Ctrl Pts',(-1.10509821673782,-0.0928409665394227,
0.204327142733961));
#28689=CARTESIAN_POINT('Ctrl Pts',(-1.10595102243643,-0.0762225747374254,
0.199591971170104));
#28690=CARTESIAN_POINT('Ctrl Pts',(-1.10653577764992,-0.0595300000000001,
0.196295654879792));
#28691=CARTESIAN_POINT('',(-1.123812,-0.05953,1.37627276864339E-16));
#28692=CARTESIAN_POINT('Origin',(0.,-0.05953,0.));
#28693=CARTESIAN_POINT('',(-1.123812,-0.35718,1.37627276864339E-16));
#28694=CARTESIAN_POINT('',(-1.123812,-0.208355,1.37627276864339E-16));
#28695=CARTESIAN_POINT('Origin',(0.,-0.35718,0.));
#28696=CARTESIAN_POINT('',(-1.10653577764992,-0.05953,-0.196295654879793));
#28697=CARTESIAN_POINT('Origin',(0.,-0.05953,0.));
#28698=CARTESIAN_POINT('',(-0.843383895613249,-0.05953,-0.742736168477219));
#28699=CARTESIAN_POINT('Ctrl Pts',(-1.10653577764992,-0.0595300000000001,
-0.196295654879792));
#28700=CARTESIAN_POINT('Ctrl Pts',(-1.10595102243643,-0.0762225747374255,
-0.199591971170104));
#28701=CARTESIAN_POINT('Ctrl Pts',(-1.10509821673782,-0.0928409665394228,
-0.204327142733962));
#28702=CARTESIAN_POINT('Ctrl Pts',(-1.10139388218929,-0.144299303100741,
-0.22376314604679));
#28703=CARTESIAN_POINT('Ctrl Pts',(-1.09728268713976,-0.177024326825049,
-0.243890930799338));
#28704=CARTESIAN_POINT('Ctrl Pts',(-1.08664560412098,-0.227269801620063,
-0.287406530683753));
#28705=CARTESIAN_POINT('Ctrl Pts',(-1.0788165083757,-0.251265615809407,
-0.316022600643821));
#28706=CARTESIAN_POINT('Ctrl Pts',(-1.06356957703048,-0.279889827963178,
-0.363699428370918));
#28707=CARTESIAN_POINT('Ctrl Pts',(-1.05494634094458,-0.290879136862659,
-0.388295406390235));
#28708=CARTESIAN_POINT('Ctrl Pts',(-1.03504317708586,-0.305251990234488,
-0.438600874831839));
#28709=CARTESIAN_POINT('Ctrl Pts',(-1.02374168767024,-0.308638795020976,
-0.46430090015576));
#28710=CARTESIAN_POINT('Ctrl Pts',(-1.00129756308006,-0.308638795020976,
-0.510906605094603));
#28711=CARTESIAN_POINT('Ctrl Pts',(-0.988250837578047,-0.305251990234488,
-0.535766169015486));
#28712=CARTESIAN_POINT('Ctrl Pts',(-0.961329858300736,-0.290879136862659,
-0.582692035672022));
#28713=CARTESIAN_POINT('Ctrl Pts',(-0.947476448101718,-0.279889827963178,
-0.604769294586516));
#28714=CARTESIAN_POINT('Ctrl Pts',(-0.919707509403859,-0.251265615809407,
-0.646415841396062));
#28715=CARTESIAN_POINT('Ctrl Pts',(-0.902215926359523,-0.227269801620064,
-0.670378702718353));
#28716=CARTESIAN_POINT('Ctrl Pts',(-0.87482617317514,-0.177024326825049,
-0.705826641853758));
#28717=CARTESIAN_POINT('Ctrl Pts',(-0.861652925570091,-0.144299303100741,
-0.721590372101268));
#28718=CARTESIAN_POINT('Ctrl Pts',(-0.848766861100456,-0.0928409665394229,
-0.736604687327351));
#28719=CARTESIAN_POINT('Ctrl Pts',(-0.84559647055299,-0.0762225747374255,
-0.740223768851063));
#28720=CARTESIAN_POINT('Ctrl Pts',(-0.843383895613249,-0.0595300000000001,
-0.742736168477219));
#28721=CARTESIAN_POINT('',(-0.536443649899847,-0.05953,-0.987512846410683));
#28722=CARTESIAN_POINT('Origin',(0.,-0.05953,0.));
#28723=CARTESIAN_POINT('',(0.0548532617164172,-0.05953,-1.12247250791415));
#28724=CARTESIAN_POINT('Ctrl Pts',(-0.536443649899848,-0.0595300000000001,
-0.987512846410683));
#28725=CARTESIAN_POINT('Ctrl Pts',(-0.533501897135712,-0.0762225747374254,
-0.989110885965947));
#28726=CARTESIAN_POINT('Ctrl Pts',(-0.529268075276156,-0.0928409665394227,
-0.991396466802469));
#28727=CARTESIAN_POINT('Ctrl Pts',(-0.511762781179147,-0.144299303100741,
-1.00061845128527));
#28728=CARTESIAN_POINT('Ctrl Pts',(-0.493462957200432,-0.177024326825049,
-1.0099536580922));
#28729=CARTESIAN_POINT('Ctrl Pts',(-0.45280897844858,-0.227269801620063,
-1.02876878445619));
#28730=CARTESIAN_POINT('Ctrl Pts',(-0.425554672694337,-0.251265615809407,
-1.04048957871266));
#28731=CARTESIAN_POINT('Ctrl Pts',(-0.3787731215897,-0.279889827963178,
-1.05829506364875));
#28732=CARTESIAN_POINT('Ctrl Pts',(-0.354166711873529,-0.290879136862659,
-1.06688848765783));
#28733=CARTESIAN_POINT('Ctrl Pts',(-0.302426893214944,-0.305251990234488,
-1.08269251410343));
#28734=CARTESIAN_POINT('Ctrl Pts',(-0.275287440920027,-0.308638795020976,
-1.0898803575765));
#28735=CARTESIAN_POINT('Ctrl Pts',(-0.224855950742601,-0.308638795020976,
-1.10139101611326));
#28736=CARTESIAN_POINT('Ctrl Pts',(-0.19728546073067,-0.305251990234488,
-1.10669035995599));
#28737=CARTESIAN_POINT('Ctrl Pts',(-0.143812384801039,-0.290879136862659,
-1.11490049012186));
#28738=CARTESIAN_POINT('Ctrl Pts',(-0.117914228755037,-0.279889827963178,
-1.1178344036749));
#28739=CARTESIAN_POINT('Ctrl Pts',(-0.0680399972366989,-0.251265615809407,
-1.12208997038458));
#28740=CARTESIAN_POINT('Ctrl Pts',(-0.0383992541984084,-0.227269801620063,
-1.12335509974011));
#28741=CARTESIAN_POINT('Ctrl Pts',(0.00639229239215326,-0.177024326825049,
-1.12404235695137));
#28742=CARTESIAN_POINT('Ctrl Pts',(0.0269302585198977,-0.144299303100741,
-1.12357162229597));
#28743=CARTESIAN_POINT('Ctrl Pts',(0.04670325263426,-0.0928409665394228,
-1.12285816383385));
#28744=CARTESIAN_POINT('Ctrl Pts',(0.0515094706813703,-0.0762225747374255,
-1.12263591311425));
#28745=CARTESIAN_POINT('Ctrl Pts',(0.0548532617164176,-0.0595300000000001,
-1.12247250791414));
#28746=CARTESIAN_POINT('',(0.437601487681057,-0.05953,-1.03511272300331));
#28747=CARTESIAN_POINT('Origin',(0.,-0.05953,0.));
#28748=CARTESIAN_POINT('',(0.911784794170997,-0.05953,-0.656964154625313));
#28749=CARTESIAN_POINT('Ctrl Pts',(0.437601487681056,-0.0595300000000001,
-1.03511272300331));
#28750=CARTESIAN_POINT('Ctrl Pts',(0.440685038163619,-0.0762225747374255,
-1.03380912944435));
#28751=CARTESIAN_POINT('Ctrl Pts',(0.445111721969657,-0.0928409665394228,
-1.03192403056628));
#28752=CARTESIAN_POINT('Ctrl Pts',(0.463236132117164,-0.144299303100741,
-1.0239876538093));
#28753=CARTESIAN_POINT('Ctrl Pts',(0.481944444320713,-0.177024326825049,
-1.01550068154148));
#28754=CARTESIAN_POINT('Ctrl Pts',(0.522002043615455,-0.227269801620064,
-0.995447160474328));
#28755=CARTESIAN_POINT('Ctrl Pts',(0.548158511259203,-0.251265615809407,
-0.981446681891443));
#28756=CARTESIAN_POINT('Ctrl Pts',(0.591247219971725,-0.279889827963178,
-0.955972930713954));
#28757=CARTESIAN_POINT('Ctrl Pts',(0.613307674922609,-0.290879136862659,
-0.942092777160053));
#28758=CARTESIAN_POINT('Ctrl Pts',(0.657923009631182,-0.305251990234487,
-0.91149460735272));
#28759=CARTESIAN_POINT('Ctrl Pts',(0.680463863683393,-0.308638795020976,
-0.894757676234429));
#28760=CARTESIAN_POINT('Ctrl Pts',(0.720906778729542,-0.308638795020976,
-0.862505527716294));
#28761=CARTESIAN_POINT('Ctrl Pts',(0.742239891936899,-0.305251990234488,
-0.844254137480381));
#28762=CARTESIAN_POINT('Ctrl Pts',(0.781998747691872,-0.290879136862659,
-0.80756613568454));
#28763=CARTESIAN_POINT('Ctrl Pts',(0.800439809856112,-0.279889827963178,
-0.789147407129765));
#28764=CARTESIAN_POINT('Ctrl Pts',(0.834863020612702,-0.251265615809407,
-0.752807465209441));
#28765=CARTESIAN_POINT('Ctrl Pts',(0.854332839576145,-0.227269801620064,
-0.73042219438957));
#28766=CARTESIAN_POINT('Ctrl Pts',(0.882797231409153,-0.177024326825049,
-0.695831250979106));
#28767=CARTESIAN_POINT('Ctrl Pts',(0.895234408667242,-0.144299303100741,
-0.679480524217551));
#28768=CARTESIAN_POINT('Ctrl Pts',(0.907004864562642,-0.0928409665394228,
-0.663576540841106));
#28769=CARTESIAN_POINT('Ctrl Pts',(0.909827729890942,-0.0762225747374256,
-0.659680317203144));
#28770=CARTESIAN_POINT('Ctrl Pts',(0.911784794170998,-0.0595300000000001,
-0.656964154625312));
#28771=CARTESIAN_POINT('',(1.08212377959455,-0.05953,-0.303251606722892));
#28772=CARTESIAN_POINT('Origin',(0.,-0.05953,0.));
#28773=CARTESIAN_POINT('',(1.08212377959455,-0.05953,0.303251606722892));
#28774=CARTESIAN_POINT('Ctrl Pts',(1.08212377959455,-0.0595300000000001,
-0.303251606722892));
#28775=CARTESIAN_POINT('Ctrl Pts',(1.0830271513892,-0.0762225747374255,
-0.300028012588062));
#28776=CARTESIAN_POINT('Ctrl Pts',(1.08431331394788,-0.0928409665394228,
-0.2953917518996));
#28777=CARTESIAN_POINT('Ctrl Pts',(1.08940878963422,-0.144299303100741,
-0.276273267473431));
#28778=CARTESIAN_POINT('Ctrl Pts',(1.09443784939331,-0.177024326825049,
-0.256354979351213));
#28779=CARTESIAN_POINT('Ctrl Pts',(1.10373487993589,-0.227269801620064,
-0.212533521233765));
#28780=CARTESIAN_POINT('Ctrl Pts',(1.10909715583869,-0.251265615809407,
-0.183354415742157));
#28781=CARTESIAN_POINT('Ctrl Pts',(1.1160463456491,-0.279889827963178,-0.133783682657561));
#28782=CARTESIAN_POINT('Ctrl Pts',(1.11894887330541,-0.290879136862659,
-0.107881990270302));
#28783=CARTESIAN_POINT('Ctrl Pts',(1.12284346704144,-0.305251990234488,
-0.0539226701638766));
#28784=CARTESIAN_POINT('Ctrl Pts',(1.123812,-0.308638795020976,-0.025864214957475));
#28785=CARTESIAN_POINT('Ctrl Pts',(1.123812,-0.308638795020976,0.025864214957475));
#28786=CARTESIAN_POINT('Ctrl Pts',(1.12284346704144,-0.305251990234488,
0.0539226701638766));
#28787=CARTESIAN_POINT('Ctrl Pts',(1.11894887330541,-0.290879136862659,
0.107881990270302));
#28788=CARTESIAN_POINT('Ctrl Pts',(1.1160463456491,-0.279889827963178,0.133783682657561));
#28789=CARTESIAN_POINT('Ctrl Pts',(1.10909715583869,-0.251265615809407,
0.183354415742157));
#28790=CARTESIAN_POINT('Ctrl Pts',(1.10373487993589,-0.227269801620064,
0.212533521233765));
#28791=CARTESIAN_POINT('Ctrl Pts',(1.09443784939331,-0.177024326825049,
0.256354979351213));
#28792=CARTESIAN_POINT('Ctrl Pts',(1.08940878963422,-0.144299303100741,
0.276273267473431));
#28793=CARTESIAN_POINT('Ctrl Pts',(1.08431331394788,-0.0928409665394228,
0.2953917518996));
#28794=CARTESIAN_POINT('Ctrl Pts',(1.0830271513892,-0.0762225747374255,
0.300028012588062));
#28795=CARTESIAN_POINT('Ctrl Pts',(1.08212377959455,-0.0595300000000001,
0.303251606722892));
#28796=CARTESIAN_POINT('Origin',(0.,-0.05953,0.));
#28797=CARTESIAN_POINT('Origin',(0.,-0.05953,0.));
#28798=CARTESIAN_POINT('',(0.0589974094846122,-0.05953,1.07456964270265));
#28799=CARTESIAN_POINT('Origin',(0.,-0.05953,0.));
#28800=CARTESIAN_POINT('Origin',(-0.244773027351946,-0.05953,1.07242070340001));
#28801=CARTESIAN_POINT('Origin',(-0.244773027351946,0.,1.07242070340001));
#28802=CARTESIAN_POINT('',(-0.519393123750572,-0.05953,0.942555777842682));
#28803=CARTESIAN_POINT('Ctrl Pts',(-0.519393123750572,-0.05953,0.942555777842682));
#28804=CARTESIAN_POINT('Ctrl Pts',(-0.513714466572041,-0.0925528133349865,
0.945684988399766));
#28805=CARTESIAN_POINT('Ctrl Pts',(-0.503136848051455,-0.124911173756694,
0.951483858396181));
#28806=CARTESIAN_POINT('Ctrl Pts',(-0.47593627990192,-0.177924977804098,
0.965323333309091));
#28807=CARTESIAN_POINT('Ctrl Pts',(-0.460931856495794,-0.199697230012983,
0.972669835243841));
#28808=CARTESIAN_POINT('Ctrl Pts',(-0.426157505475872,-0.237895043532788,
0.988400002689705));
#28809=CARTESIAN_POINT('Ctrl Pts',(-0.406380688682952,-0.254319232363049,
0.996771768218699));
#28810=CARTESIAN_POINT('Ctrl Pts',(-0.364750145543744,-0.28018331644634,
1.01272583306292));
#28811=CARTESIAN_POINT('Ctrl Pts',(-0.340838910881557,-0.29104845371857,
1.02112815447116));
#28812=CARTESIAN_POINT('Ctrl Pts',(-0.290495481564827,-0.30527573347708,
1.036574285215));
#28813=CARTESIAN_POINT('Ctrl Pts',(-0.264056468041074,-0.308638795020976,
1.04359501395068));
#28814=CARTESIAN_POINT('Ctrl Pts',(-0.214892249704082,-0.308638795020976,
1.05481642595959));
#28815=CARTESIAN_POINT('Ctrl Pts',(-0.188025341585962,-0.30527573347708,
1.05996242598502));
#28816=CARTESIAN_POINT('Ctrl Pts',(-0.135965654106109,-0.29104845371857,
1.06788913840721));
#28817=CARTESIAN_POINT('Ctrl Pts',(-0.110776745452494,-0.28018331644634,
1.07069360430242));
#28818=CARTESIAN_POINT('Ctrl Pts',(-0.0663467128214646,-0.254319232363049,
1.07438230428002));
#28819=CARTESIAN_POINT('Ctrl Pts',(-0.0448960436540983,-0.237895043532788,
1.07542044338697));
#28820=CARTESIAN_POINT('Ctrl Pts',(-0.00674037211528124,-0.199697230012983,
1.07633607767727));
#28821=CARTESIAN_POINT('Ctrl Pts',(0.00996567398334777,-0.177924977804098,
1.07622728347683));
#28822=CARTESIAN_POINT('Ctrl Pts',(0.0404772621979741,-0.124911173756694,
1.07556023164702));
#28823=CARTESIAN_POINT('Ctrl Pts',(0.0525234025782719,-0.0925528133349865,
1.07492508698591));
#28824=CARTESIAN_POINT('Ctrl Pts',(0.0589974094846124,-0.05953,1.07456964270265));
#28825=CARTESIAN_POINT('Origin',(-0.244773027351946,-0.05953,1.07242070340001));
#28826=CARTESIAN_POINT('Origin',(0.,-0.05953,0.));
#28827=CARTESIAN_POINT('',(-0.803348093619616,-0.05953,0.716109245731214));
#28828=CARTESIAN_POINT('Origin',(0.,-0.05953,0.));
#28829=CARTESIAN_POINT('Origin',(-0.991065754692661,-0.05953,0.477272113029314));
#28830=CARTESIAN_POINT('Origin',(-0.991065754692661,0.,0.477272113029314));
#28831=CARTESIAN_POINT('',(-1.06075609691358,-0.05953,0.181596019242328));
#28832=CARTESIAN_POINT('Ctrl Pts',(-1.06075609691358,-0.05953,0.181596019242328));
#28833=CARTESIAN_POINT('Ctrl Pts',(-1.05966202740332,-0.0925528133349865,
0.187986803072856));
#28834=CARTESIAN_POINT('Ctrl Pts',(-1.05760072925372,-0.124911173756694,
0.199872254546857));
#28835=CARTESIAN_POINT('Ctrl Pts',(-1.05146158959546,-0.177924977804098,
0.22976728653846));
#28836=CARTESIAN_POINT('Ctrl Pts',(-1.04785021111757,-0.199697230012983,
0.246078686169301));
#28837=CARTESIAN_POINT('Ctrl Pts',(-1.03846709802406,-0.237895043532788,
0.283073967563097));
#28838=CARTESIAN_POINT('Ctrl Pts',(-1.03268176429485,-0.254319232363049,
0.303755815985685));
#28839=CARTESIAN_POINT('Ctrl Pts',(-1.01919893537026,-0.28018331644634,
0.346251081972725));
#28840=CARTESIAN_POINT('Ctrl Pts',(-1.01085972381132,-0.29104845371857,
0.370184399726282));
#28841=CARTESIAN_POINT('Ctrl Pts',(-0.99154738033959,-0.30527573347708,
0.419174982698463));
#28842=CARTESIAN_POINT('Ctrl Pts',(-0.980551951791748,-0.308638795020976,
0.444223188605045));
#28843=CARTESIAN_POINT('Ctrl Pts',(-0.958671816228589,-0.308638795020976,
0.489657758261848));
#28844=CARTESIAN_POINT('Ctrl Pts',(-0.945943877838127,-0.30527573347708,
0.51387163140139));
#28845=CARTESIAN_POINT('Ctrl Pts',(-0.91968254693063,-0.29104845371857,
0.559515758398093));
#28846=CARTESIAN_POINT('Ctrl Pts',(-0.906170138993533,-0.28018331644634,
0.580957796077825));
#28847=CARTESIAN_POINT('Ctrl Pts',(-0.8813524085237,-0.254319232363049,
0.617994461173994));
#28848=CARTESIAN_POINT('Ctrl Pts',(-0.868789784891799,-0.237895043532788,
0.635412538795143));
#28849=CARTESIAN_POINT('Ctrl Pts',(-0.845715984518854,-0.199697230012983,
0.66581473268113));
#28850=CARTESIAN_POINT('Ctrl Pts',(-0.835214876415962,-0.177924977804098,
0.678808213394124));
#28851=CARTESIAN_POINT('Ctrl Pts',(-0.815669690204649,-0.124911173756694,
0.702247233627224));
#28852=CARTESIAN_POINT('Ctrl Pts',(-0.807662468433796,-0.0925528133349865,
0.711269279199861));
#28853=CARTESIAN_POINT('Ctrl Pts',(-0.803348093619616,-0.05953,0.716109245731214));
#28854=CARTESIAN_POINT('Origin',(-0.991065754692661,-0.05953,0.477272113029314));
#28855=CARTESIAN_POINT('Origin',(0.,-0.05953,0.));
#28856=CARTESIAN_POINT('',(-1.076188,-0.05953,1.31795018948079E-16));
#28857=CARTESIAN_POINT('Origin',(0.,-0.05953,0.));
#28858=CARTESIAN_POINT('',(-1.06075609691358,-0.05953,-0.181596019242328));
#28859=CARTESIAN_POINT('Origin',(0.,-0.05953,0.));
#28860=CARTESIAN_POINT('Origin',(-0.991065754692661,-0.05953,-0.477272113029314));
#28861=CARTESIAN_POINT('Origin',(-0.991065754692661,0.,-0.477272113029314));
#28862=CARTESIAN_POINT('',(-0.803348093619616,-0.05953,-0.716109245731215));
#28863=CARTESIAN_POINT('Ctrl Pts',(-0.803348093619616,-0.05953,-0.716109245731215));
#28864=CARTESIAN_POINT('Ctrl Pts',(-0.807662468433795,-0.0925528133349865,
-0.711269279199862));
#28865=CARTESIAN_POINT('Ctrl Pts',(-0.815669690204649,-0.124911173756694,
-0.702247233627224));
#28866=CARTESIAN_POINT('Ctrl Pts',(-0.835214876415962,-0.177924977804098,
-0.678808213394124));
#28867=CARTESIAN_POINT('Ctrl Pts',(-0.845715984518854,-0.199697230012983,
-0.66581473268113));
#28868=CARTESIAN_POINT('Ctrl Pts',(-0.868789784891799,-0.237895043532788,
-0.635412538795143));
#28869=CARTESIAN_POINT('Ctrl Pts',(-0.8813524085237,-0.254319232363049,
-0.617994461173994));
#28870=CARTESIAN_POINT('Ctrl Pts',(-0.906170138993533,-0.28018331644634,
-0.580957796077826));
#28871=CARTESIAN_POINT('Ctrl Pts',(-0.91968254693063,-0.29104845371857,
-0.559515758398093));
#28872=CARTESIAN_POINT('Ctrl Pts',(-0.945943877838127,-0.30527573347708,
-0.51387163140139));
#28873=CARTESIAN_POINT('Ctrl Pts',(-0.958671816228589,-0.308638795020976,
-0.489657758261848));
#28874=CARTESIAN_POINT('Ctrl Pts',(-0.980551951791748,-0.308638795020976,
-0.444223188605045));
#28875=CARTESIAN_POINT('Ctrl Pts',(-0.99154738033959,-0.30527573347708,
-0.419174982698463));
#28876=CARTESIAN_POINT('Ctrl Pts',(-1.01085972381132,-0.29104845371857,
-0.370184399726282));
#28877=CARTESIAN_POINT('Ctrl Pts',(-1.01919893537026,-0.28018331644634,
-0.346251081972725));
#28878=CARTESIAN_POINT('Ctrl Pts',(-1.03268176429485,-0.254319232363049,
-0.303755815985685));
#28879=CARTESIAN_POINT('Ctrl Pts',(-1.03846709802406,-0.237895043532788,
-0.283073967563097));
#28880=CARTESIAN_POINT('Ctrl Pts',(-1.04785021111757,-0.199697230012983,
-0.246078686169302));
#28881=CARTESIAN_POINT('Ctrl Pts',(-1.05146158959546,-0.177924977804098,
-0.229767286538461));
#28882=CARTESIAN_POINT('Ctrl Pts',(-1.05760072925372,-0.124911173756694,
-0.199872254546858));
#28883=CARTESIAN_POINT('Ctrl Pts',(-1.05966202740332,-0.0925528133349864,
-0.187986803072857));
#28884=CARTESIAN_POINT('Ctrl Pts',(-1.06075609691358,-0.05953,-0.181596019242328));
#28885=CARTESIAN_POINT('Origin',(-0.991065754692661,-0.05953,-0.477272113029314));
#28886=CARTESIAN_POINT('Origin',(0.,-0.05953,0.));
#28887=CARTESIAN_POINT('',(-0.519393123750572,-0.05953,-0.942555777842682));
#28888=CARTESIAN_POINT('Origin',(0.,-0.05953,0.));
#28889=CARTESIAN_POINT('Origin',(-0.244773027351946,-0.05953,-1.07242070340001));
#28890=CARTESIAN_POINT('Origin',(-0.244773027351946,0.,-1.07242070340001));
#28891=CARTESIAN_POINT('',(0.0589974094846125,-0.05953,-1.07456964270265));
#28892=CARTESIAN_POINT('Ctrl Pts',(0.0589974094846127,-0.05953,-1.07456964270265));
#28893=CARTESIAN_POINT('Ctrl Pts',(0.0525234025782722,-0.0925528133349865,
-1.07492508698591));
#28894=CARTESIAN_POINT('Ctrl Pts',(0.0404772621979744,-0.124911173756694,
-1.07556023164702));
#28895=CARTESIAN_POINT('Ctrl Pts',(0.0099656739833481,-0.177924977804098,
-1.07622728347683));
#28896=CARTESIAN_POINT('Ctrl Pts',(-0.00674037211528096,-0.199697230012983,
-1.07633607767727));
#28897=CARTESIAN_POINT('Ctrl Pts',(-0.044896043654098,-0.237895043532788,
-1.07542044338697));
#28898=CARTESIAN_POINT('Ctrl Pts',(-0.0663467128214644,-0.254319232363049,
-1.07438230428002));
#28899=CARTESIAN_POINT('Ctrl Pts',(-0.110776745452493,-0.28018331644634,
-1.07069360430242));
#28900=CARTESIAN_POINT('Ctrl Pts',(-0.135965654106109,-0.29104845371857,
-1.06788913840721));
#28901=CARTESIAN_POINT('Ctrl Pts',(-0.188025341585962,-0.30527573347708,
-1.05996242598502));
#28902=CARTESIAN_POINT('Ctrl Pts',(-0.214892249704082,-0.308638795020976,
-1.05481642595959));
#28903=CARTESIAN_POINT('Ctrl Pts',(-0.264056468041074,-0.308638795020976,
-1.04359501395068));
#28904=CARTESIAN_POINT('Ctrl Pts',(-0.290495481564827,-0.30527573347708,
-1.036574285215));
#28905=CARTESIAN_POINT('Ctrl Pts',(-0.340838910881557,-0.291048453718569,
-1.02112815447116));
#28906=CARTESIAN_POINT('Ctrl Pts',(-0.364750145543744,-0.28018331644634,
-1.01272583306292));
#28907=CARTESIAN_POINT('Ctrl Pts',(-0.406380688682952,-0.254319232363049,
-0.996771768218699));
#28908=CARTESIAN_POINT('Ctrl Pts',(-0.426157505475872,-0.237895043532788,
-0.988400002689705));
#28909=CARTESIAN_POINT('Ctrl Pts',(-0.460931856495794,-0.199697230012983,
-0.972669835243841));
#28910=CARTESIAN_POINT('Ctrl Pts',(-0.475936279901919,-0.177924977804098,
-0.965323333309091));
#28911=CARTESIAN_POINT('Ctrl Pts',(-0.503136848051454,-0.124911173756694,
-0.951483858396181));
#28912=CARTESIAN_POINT('Ctrl Pts',(-0.513714466572041,-0.0925528133349865,
-0.945684988399766));
#28913=CARTESIAN_POINT('Ctrl Pts',(-0.519393123750572,-0.05953,-0.942555777842682));
#28914=CARTESIAN_POINT('Origin',(-0.244773027351946,-0.05953,-1.07242070340001));
#28915=CARTESIAN_POINT('Origin',(0.,-0.05953,0.));
#28916=CARTESIAN_POINT('',(0.413083465285518,-0.05953,-0.993751811093549));
#28917=CARTESIAN_POINT('Origin',(0.,-0.05953,0.));
#28918=CARTESIAN_POINT('Origin',(0.685838782044607,-0.05953,-0.860014630714833));
#28919=CARTESIAN_POINT('Origin',(0.685838782044607,0.,-0.860014630714833));
#28920=CARTESIAN_POINT('',(0.876916659919095,-0.05953,-0.623857181492959));
#28921=CARTESIAN_POINT('Ctrl Pts',(0.876916659919095,-0.05953,-0.623857181492958));
#28922=CARTESIAN_POINT('Ctrl Pts',(0.873158080166742,-0.0925528133349865,
-0.62914037979579));
#28923=CARTESIAN_POINT('Ctrl Pts',(0.866144010579847,-0.124911173756694,
-0.638954437806245));
#28924=CARTESIAN_POINT('Ctrl Pts',(0.847641868610495,-0.177924977804098,
-0.663225258065736));
#28925=CARTESIAN_POINT('Ctrl Pts',(0.837310877969633,-0.199697230012983,
-0.676354402927683));
#28926=CARTESIAN_POINT('Ctrl Pts',(0.81280533416753,-0.237895043532788,
-0.705614819529209));
#28927=CARTESIAN_POINT('Ctrl Pts',(0.798619410861634,-0.254319232363049,
-0.721738358858166));
#28928=CARTESIAN_POINT('Ctrl Pts',(0.768033796848072,-0.28018331644634,
-0.754175290318038));
#28929=CARTESIAN_POINT('Ctrl Pts',(0.750136149454208,-0.29104845371857,
-0.772120216227122));
#28930=CARTESIAN_POINT('Ctrl Pts',(0.711480111898423,-0.30527573347708,
-0.807879894508811));
#28931=CARTESIAN_POINT('Ctrl Pts',(0.690705563850638,-0.308638795020976,
-0.825676810575913));
#28932=CARTESIAN_POINT('Ctrl Pts',(0.651278921914856,-0.308638795020976,
-0.857118508332695));
#28933=CARTESIAN_POINT('Ctrl Pts',(0.629305439856167,-0.30527573347708,
-0.873412008702649));
#28934=CARTESIAN_POINT('Ctrl Pts',(0.585840553788742,-0.29104845371857,
-0.903141581680914));
#28935=CARTESIAN_POINT('Ctrl Pts',(0.564362943424239,-0.28018331644634,
-0.916597376014514));
#28936=CARTESIAN_POINT('Ctrl Pts',(0.525933334162556,-0.254319232363049,
-0.939198248544427));
#28937=CARTESIAN_POINT('Ctrl Pts',(0.507057380724533,-0.237895043532788,
-0.949440676105255));
#28938=CARTESIAN_POINT('Ctrl Pts',(0.473077587363686,-0.199697230012983,
-0.966820759530997));
#28939=CARTESIAN_POINT('Ctrl Pts',(0.457978755888596,-0.177924977804098,
-0.973971221090534));
#28940=CARTESIAN_POINT('Ctrl Pts',(0.430199341854858,-0.124911173756694,
-0.986608710139579));
#28941=CARTESIAN_POINT('Ctrl Pts',(0.419070565453384,-0.0925528133349865,
-0.991263089003441));
#28942=CARTESIAN_POINT('Ctrl Pts',(0.413083465285518,-0.05953,-0.993751811093549));
#28943=CARTESIAN_POINT('Origin',(0.685838782044607,-0.05953,-0.860014630714833));
#28944=CARTESIAN_POINT('Origin',(0.,-0.208355,0.));
#28945=CARTESIAN_POINT('',(-1.076188,-0.35718,1.31795018948079E-16));
#28946=CARTESIAN_POINT('Origin',(0.,-0.35718,0.));
#28947=CARTESIAN_POINT('',(-1.076188,-0.208355,1.31795018948079E-16));
#28948=CARTESIAN_POINT('',(1.03449977959455,-0.05953,0.296632461748266));
#28949=CARTESIAN_POINT('Origin',(0.,-0.05953,0.));
#28950=CARTESIAN_POINT('',(1.03449977959455,-0.05953,-0.296632461748266));
#28951=CARTESIAN_POINT('Ctrl Pts',(1.03449977959455,-0.05953,0.296632461748267));
#28952=CARTESIAN_POINT('Ctrl Pts',(1.03628691421076,-0.0925528133349865,
0.290399865505497));
#28953=CARTESIAN_POINT('Ctrl Pts',(1.03958665287714,-0.124911173756694,
0.278797079997872));
#28954=CARTESIAN_POINT('Ctrl Pts',(1.0470264474309,-0.177924977804098,0.249198913998601));
#28955=CARTESIAN_POINT('Ctrl Pts',(1.05084995891418,-0.199697230012983,
0.232935932341942));
#28956=CARTESIAN_POINT('Ctrl Pts',(1.05844771715377,-0.237895043532788,
0.195533155353269));
#28957=CARTESIAN_POINT('Ctrl Pts',(1.06220882929878,-0.254319232363049,
0.17438929156337));
#28958=CARTESIAN_POINT('Ctrl Pts',(1.06849922508772,-0.28018331644634,0.130252399648131));
#28959=CARTESIAN_POINT('Ctrl Pts',(1.07137013248666,-0.29104845371857,0.105070977154072));
#28960=CARTESIAN_POINT('Ctrl Pts',(1.07522652957392,-0.30527573347708,0.0525526752791107));
#28961=CARTESIAN_POINT('Ctrl Pts',(1.076188,-0.308638795020976,0.025214283908933));
#28962=CARTESIAN_POINT('Ctrl Pts',(1.076188,-0.308638795020976,-0.025214283908933));
#28963=CARTESIAN_POINT('Ctrl Pts',(1.07522652957392,-0.30527573347708,-0.0525526752791107));
#28964=CARTESIAN_POINT('Ctrl Pts',(1.07137013248666,-0.29104845371857,-0.105070977154072));
#28965=CARTESIAN_POINT('Ctrl Pts',(1.06849922508772,-0.28018331644634,-0.130252399648131));
#28966=CARTESIAN_POINT('Ctrl Pts',(1.06220882929878,-0.254319232363049,
-0.17438929156337));
#28967=CARTESIAN_POINT('Ctrl Pts',(1.05844771715377,-0.237895043532788,
-0.195533155353269));
#28968=CARTESIAN_POINT('Ctrl Pts',(1.05084995891418,-0.199697230012983,
-0.232935932341942));
#28969=CARTESIAN_POINT('Ctrl Pts',(1.0470264474309,-0.177924977804098,-0.249198913998601));
#28970=CARTESIAN_POINT('Ctrl Pts',(1.03958665287714,-0.124911173756694,
-0.278797079997872));
#28971=CARTESIAN_POINT('Ctrl Pts',(1.03628691421076,-0.0925528133349865,
-0.290399865505497));
#28972=CARTESIAN_POINT('Ctrl Pts',(1.03449977959455,-0.05953,-0.296632461748267));
#28973=CARTESIAN_POINT('Origin',(0.,-0.05953,0.));
#28974=CARTESIAN_POINT('Origin',(0.,-0.05953,0.));
#28975=CARTESIAN_POINT('Origin',(1.1,-0.05953,0.));
#28976=CARTESIAN_POINT('Origin',(1.1,0.,0.));
#28977=CARTESIAN_POINT('Origin',(1.1,-0.05953,0.));
#28978=CARTESIAN_POINT('Origin',(0.,-0.35718,0.));
#28979=CARTESIAN_POINT('Origin',(0.,-0.05953,0.));
#43415=UNCERTAINTY_MEASURE_WITH_UNIT(LENGTH_MEASURE(0.001),#43522,
'DISTANCE_ACCURACY_VALUE',
'Maximum model space distance between geometric entities at asserted c
onnectivities');
#43453=UNCERTAINTY_MEASURE_WITH_UNIT(LENGTH_MEASURE(0.001),#43522,
'DISTANCE_ACCURACY_VALUE',
'Maximum model space distance between geometric entities at asserted c
onnectivities');
#43483=(
GEOMETRIC_REPRESENTATION_CONTEXT(3)
GLOBAL_UNCERTAINTY_ASSIGNED_CONTEXT((#43415))
GLOBAL_UNIT_ASSIGNED_CONTEXT((#43522,#43524,#43525))
REPRESENTATION_CONTEXT('','3D')
);
#43521=(
GEOMETRIC_REPRESENTATION_CONTEXT(3)
GLOBAL_UNCERTAINTY_ASSIGNED_CONTEXT((#43453))
GLOBAL_UNIT_ASSIGNED_CONTEXT((#43522,#43524,#43525))
REPRESENTATION_CONTEXT('','3D')
);
#43522=(
LENGTH_UNIT()
NAMED_UNIT(*)
SI_UNIT(.CENTI.,.METRE.)
);
#43524=(
NAMED_UNIT(*)
PLANE_ANGLE_UNIT()
SI_UNIT($,.RADIAN.)
);
#43525=(
NAMED_UNIT(*)
SI_UNIT($,.STERADIAN.)
SOLID_ANGLE_UNIT()
);
#43555=SHAPE_DEFINITION_REPRESENTATION(#43622,#43823);
#43622=PRODUCT_DEFINITION_SHAPE('',$,#43891);
#43823=SHAPE_REPRESENTATION('',(#20048),#43483);
#43861=PRODUCT_DEFINITION_CONTEXT('part definition',#44064,'design');
#43891=PRODUCT_DEFINITION('Cage','Cage',#43958,#43861);
#43958=PRODUCT_DEFINITION_FORMATION('',$,#44095);
#44064=APPLICATION_CONTEXT(
'Core Data for Automotive Mechanical Design Process');
#44065=PRODUCT_CONTEXT('part definition',#44064,'mechanical');
#44095=PRODUCT('Cage','Cage','Cage',(#44065));
#44196=COLOUR_RGB('Grey',0.48,0.52,0.57);
#44197=FILL_AREA_STYLE_COLOUR('',#44196);
#44198=FILL_AREA_STYLE('',(#44197));
#44199=SURFACE_STYLE_FILL_AREA(#44198);
#44200=SURFACE_SIDE_STYLE('',(#44199));
#44201=SURFACE_STYLE_USAGE(.BOTH.,#44200);
#44202=PRESENTATION_STYLE_ASSIGNMENT((#44201));
ENDSEC;
END-ISO-10303-21;
